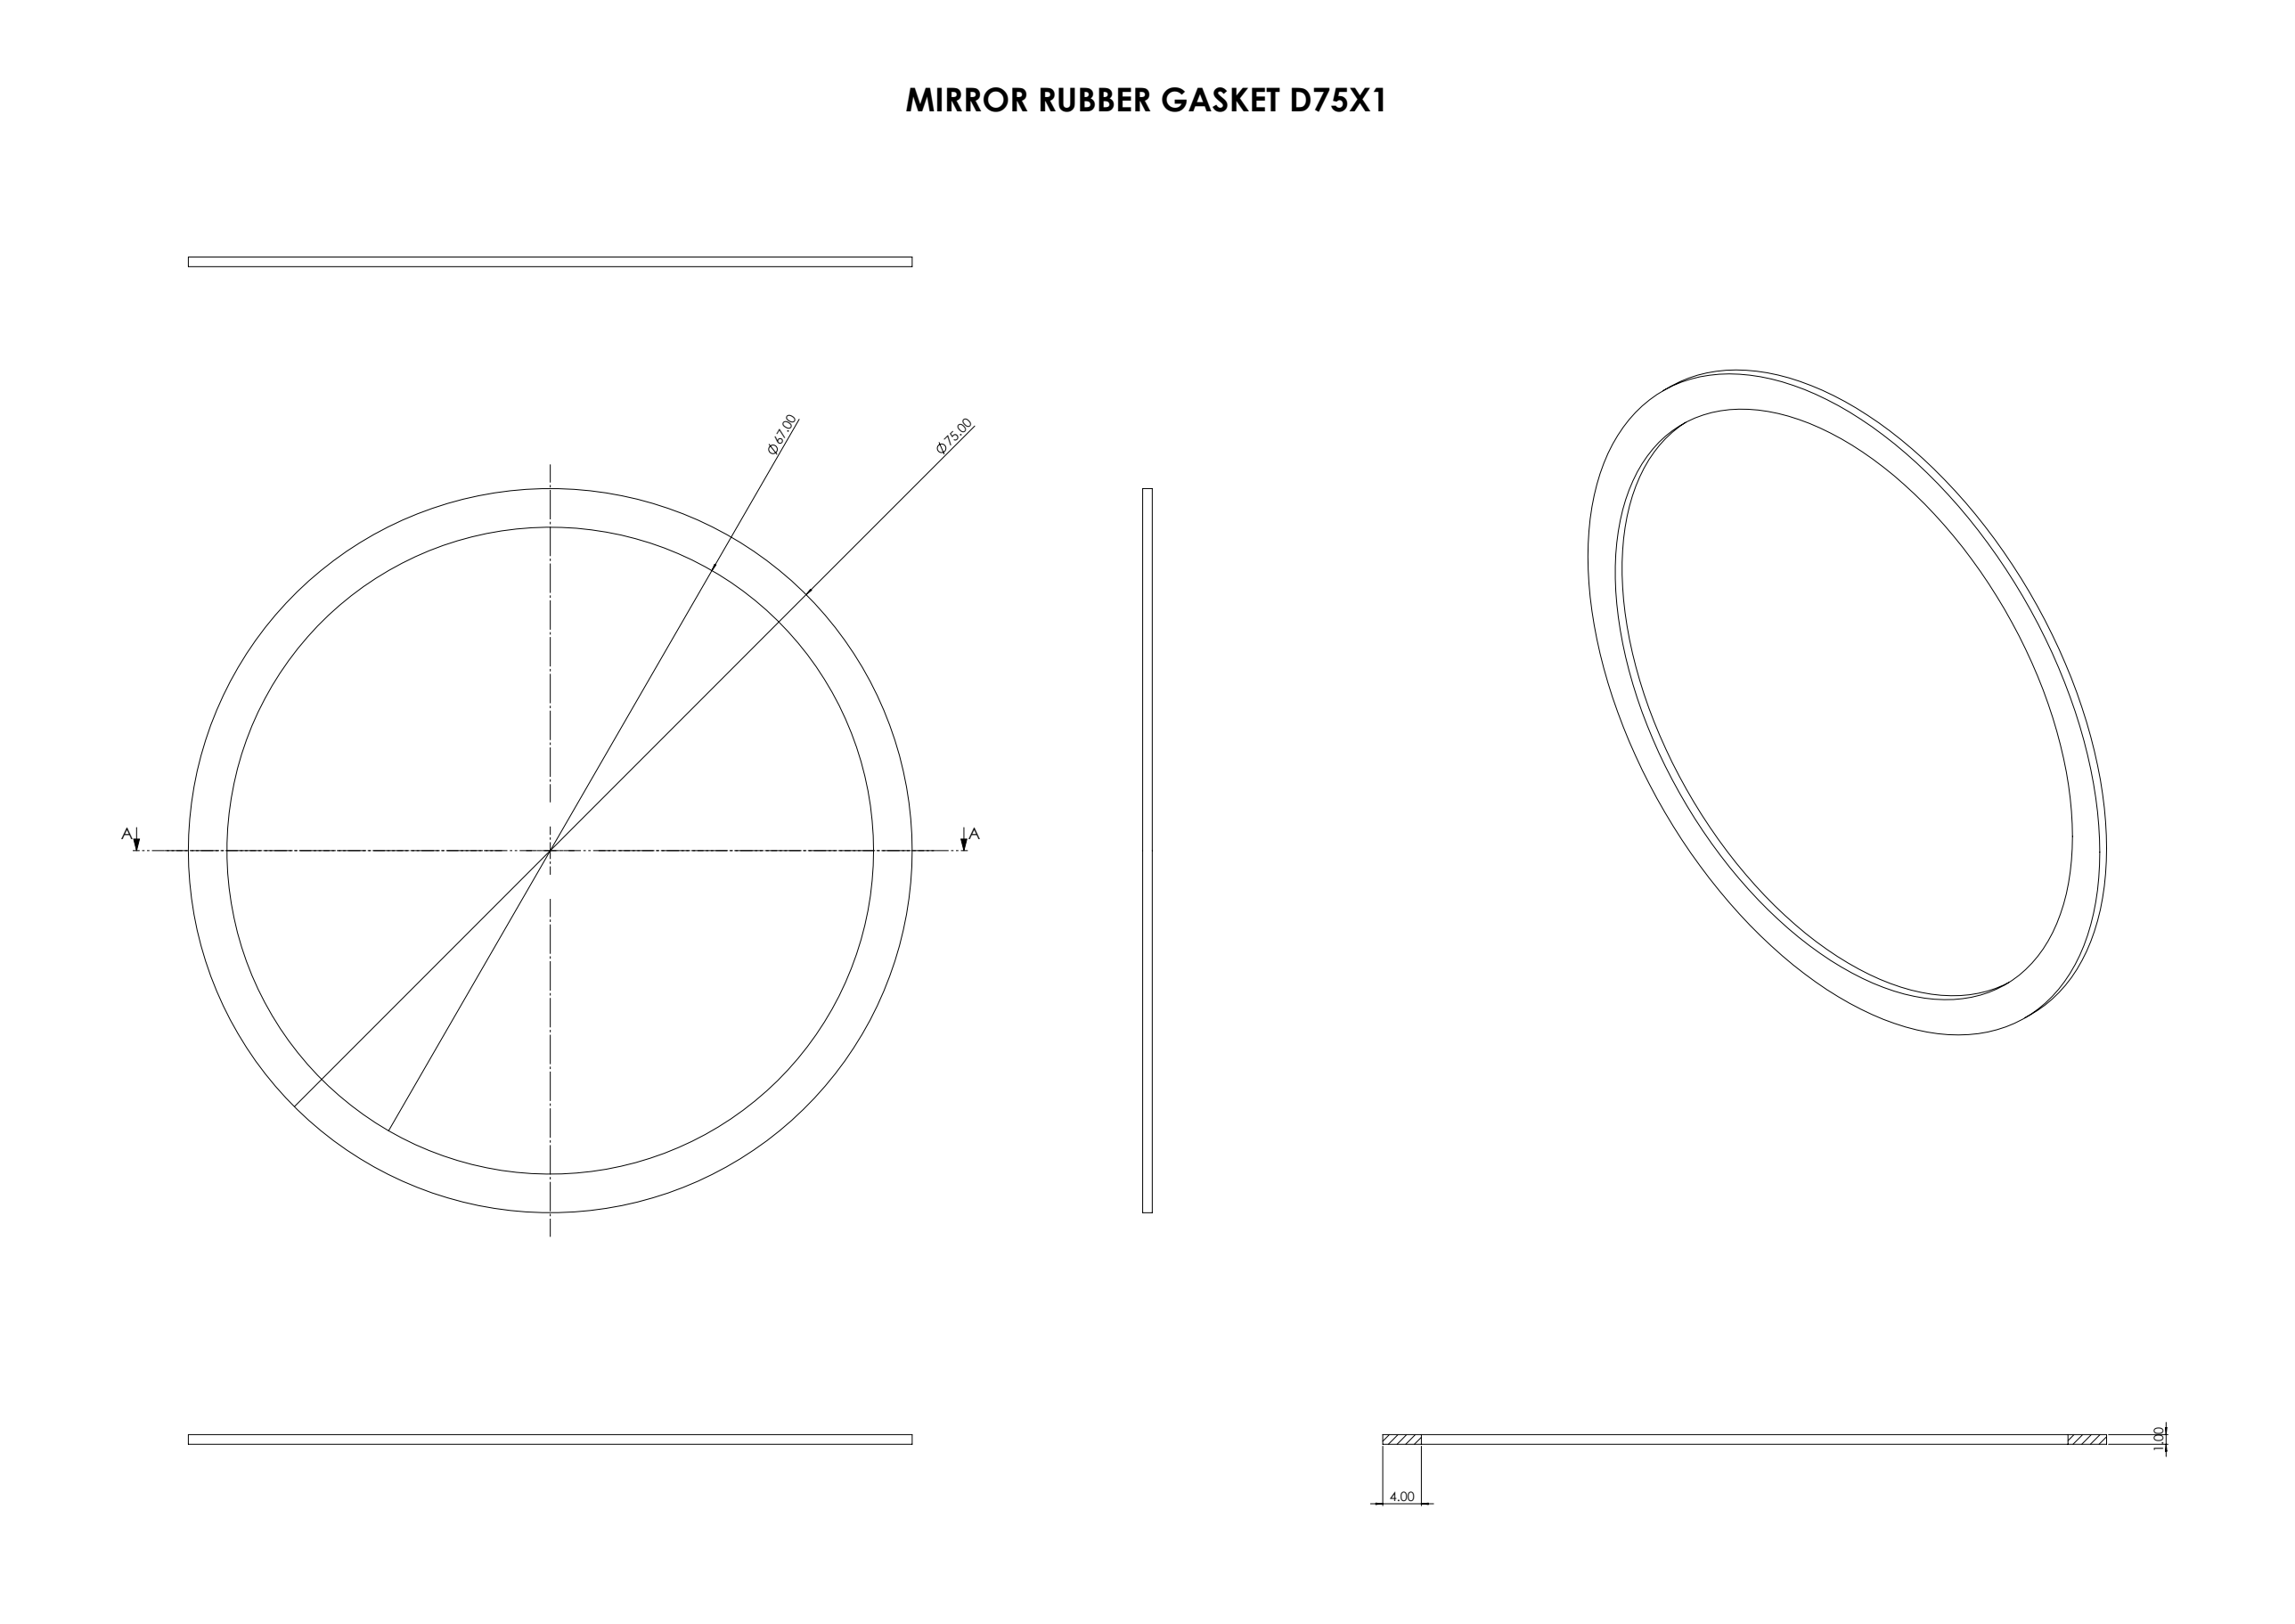
ISO-10303-21;
HEADER;
/* Generated by software containing ST-Developer
 * from STEP Tools, Inc. (www.steptools.com) 
 */

FILE_DESCRIPTION(
/* description */ (''),
/* implementation_level */ '2;1');

FILE_NAME(
/* name */ '08_Mirror_Rubber_Gasket_D75x1.step',
/* time_stamp */ '2026-10-19T22:59:19-07:00',
/* author */ (''),
/* organization */ (''),
/* preprocessor_version */ 'ST-DEVELOPER v20.2',
/* originating_system */ 'Autodesk Translation Framework v15.15.0.0',
/* authorisation */ '');

FILE_SCHEMA (('AUTOMOTIVE_DESIGN { 1 0 10303 214 3 1 1 }'));
ENDSEC;

DATA;
#10=MECHANICAL_DESIGN_GEOMETRIC_PRESENTATION_REPRESENTATION('',(#920),#53650);
#888=SHAPE_REPRESENTATION_RELATIONSHIP('SRR','None',#53733,#904);
#904=ADVANCED_BREP_SHAPE_REPRESENTATION('',(#936),#53643);
#920=STYLED_ITEM('',(#53965),#936);
#936=MANIFOLD_SOLID_BREP('Gasket',#23312);
#1044=CYLINDRICAL_SURFACE('',#24522,3.35);
#1045=CYLINDRICAL_SURFACE('',#24527,3.75);
#1410=FACE_BOUND('',#4277,.T.);
#1411=FACE_BOUND('',#4280,.T.);
#1755=PLANE('',#24525);
#1756=PLANE('',#24529);
#2814=FACE_OUTER_BOUND('',#4275,.T.);
#2815=FACE_OUTER_BOUND('',#4276,.T.);
#2816=FACE_OUTER_BOUND('',#4278,.T.);
#2817=FACE_OUTER_BOUND('',#4279,.T.);
#4275=EDGE_LOOP('',(#17615,#17616,#17617,#17618));
#4276=EDGE_LOOP('',(#17619));
#4277=EDGE_LOOP('',(#17620));
#4278=EDGE_LOOP('',(#17621,#17622,#17623,#17624));
#4279=EDGE_LOOP('',(#17625));
#4280=EDGE_LOOP('',(#17626));
#5502=CIRCLE('',#24523,3.35);
#5503=CIRCLE('',#24524,3.35);
#5504=CIRCLE('',#24526,3.75);
#5505=CIRCLE('',#24528,3.75);
#6636=LINE('',#35972,#8481);
#6637=LINE('',#35980,#8482);
#8481=VECTOR('',#28494,3.35);
#8482=VECTOR('',#28505,3.75);
#10333=VERTEX_POINT('',#35969);
#10334=VERTEX_POINT('',#35971);
#10335=VERTEX_POINT('',#35975);
#10336=VERTEX_POINT('',#35978);
#12985=EDGE_CURVE('',#10333,#10333,#5502,.T.);
#12986=EDGE_CURVE('',#10333,#10334,#6636,.T.);
#12987=EDGE_CURVE('',#10334,#10334,#5503,.T.);
#12988=EDGE_CURVE('',#10335,#10335,#5504,.T.);
#12989=EDGE_CURVE('',#10336,#10336,#5505,.T.);
#12990=EDGE_CURVE('',#10336,#10335,#6637,.T.);
#17615=ORIENTED_EDGE('',*,*,#12985,.T.);
#17616=ORIENTED_EDGE('',*,*,#12986,.T.);
#17617=ORIENTED_EDGE('',*,*,#12987,.F.);
#17618=ORIENTED_EDGE('',*,*,#12986,.F.);
#17619=ORIENTED_EDGE('',*,*,#12988,.F.);
#17620=ORIENTED_EDGE('',*,*,#12987,.T.);
#17621=ORIENTED_EDGE('',*,*,#12989,.F.);
#17622=ORIENTED_EDGE('',*,*,#12990,.T.);
#17623=ORIENTED_EDGE('',*,*,#12988,.T.);
#17624=ORIENTED_EDGE('',*,*,#12990,.F.);
#17625=ORIENTED_EDGE('',*,*,#12989,.T.);
#17626=ORIENTED_EDGE('',*,*,#12985,.F.);
#22553=ADVANCED_FACE('',(#2814),#1044,.F.);
#22554=ADVANCED_FACE('',(#2815,#1410),#1755,.T.);
#22555=ADVANCED_FACE('',(#2816),#1045,.T.);
#22556=ADVANCED_FACE('',(#2817,#1411),#1756,.T.);
#23312=CLOSED_SHELL('',(#22553,#22554,#22555,#22556));
#24521=AXIS2_PLACEMENT_3D('',#35967,#28488,#28489);
#24522=AXIS2_PLACEMENT_3D('',#35968,#28490,#28491);
#24523=AXIS2_PLACEMENT_3D('',#35970,#28492,#28493);
#24524=AXIS2_PLACEMENT_3D('',#35973,#28495,#28496);
#24525=AXIS2_PLACEMENT_3D('',#35974,#28497,#28498);
#24526=AXIS2_PLACEMENT_3D('',#35976,#28499,#28500);
#24527=AXIS2_PLACEMENT_3D('',#35977,#28501,#28502);
#24528=AXIS2_PLACEMENT_3D('',#35979,#28503,#28504);
#24529=AXIS2_PLACEMENT_3D('',#35981,#28506,#28507);
#28488=DIRECTION('axis',(0.,0.,1.));
#28489=DIRECTION('refdir',(1.,0.,0.));
#28490=DIRECTION('center_axis',(0.,0.,1.));
#28491=DIRECTION('ref_axis',(1.,0.,0.));
#28492=DIRECTION('center_axis',(0.,0.,1.));
#28493=DIRECTION('ref_axis',(1.,0.,0.));
#28494=DIRECTION('',(0.,0.,-1.));
#28495=DIRECTION('center_axis',(0.,0.,1.));
#28496=DIRECTION('ref_axis',(1.,0.,0.));
#28497=DIRECTION('center_axis',(0.,0.,-1.));
#28498=DIRECTION('ref_axis',(-1.,0.,0.));
#28499=DIRECTION('center_axis',(0.,0.,1.));
#28500=DIRECTION('ref_axis',(1.,0.,0.));
#28501=DIRECTION('center_axis',(0.,0.,1.));
#28502=DIRECTION('ref_axis',(1.,0.,0.));
#28503=DIRECTION('center_axis',(0.,0.,1.));
#28504=DIRECTION('ref_axis',(1.,0.,0.));
#28505=DIRECTION('',(0.,0.,-1.));
#28506=DIRECTION('center_axis',(0.,0.,1.));
#28507=DIRECTION('ref_axis',(1.,0.,0.));
#35967=CARTESIAN_POINT('',(0.,0.,0.));
#35968=CARTESIAN_POINT('Origin',(0.,0.,0.05));
#35969=CARTESIAN_POINT('',(-3.35,-4.10256677714363E-16,0.1));
#35970=CARTESIAN_POINT('Origin',(0.,0.,0.1));
#35971=CARTESIAN_POINT('',(-3.35,-4.10256677714363E-16,0.));
#35972=CARTESIAN_POINT('',(-3.35,-4.10256677714363E-16,0.05));
#35973=CARTESIAN_POINT('Origin',(0.,0.,0.));
#35974=CARTESIAN_POINT('Origin',(3.75,0.,0.));
#35975=CARTESIAN_POINT('',(-3.75,-4.59242549680257E-16,0.));
#35976=CARTESIAN_POINT('Origin',(0.,0.,0.));
#35977=CARTESIAN_POINT('Origin',(0.,0.,0.05));
#35978=CARTESIAN_POINT('',(-3.75,-4.59242549680257E-16,0.1));
#35979=CARTESIAN_POINT('Origin',(0.,0.,0.1));
#35980=CARTESIAN_POINT('',(-3.75,-4.59242549680257E-16,0.05));
#35981=CARTESIAN_POINT('Origin',(3.35,0.,0.1));
#53625=UNCERTAINTY_MEASURE_WITH_UNIT(LENGTH_MEASURE(0.001),#53651,
'DISTANCE_ACCURACY_VALUE',
'Maximum model space distance between geometric entities at asserted c
onnectivities');
#53632=UNCERTAINTY_MEASURE_WITH_UNIT(LENGTH_MEASURE(0.001),#53651,
'DISTANCE_ACCURACY_VALUE',
'Maximum model space distance between geometric entities at asserted c
onnectivities');
#53643=(
GEOMETRIC_REPRESENTATION_CONTEXT(3)
GLOBAL_UNCERTAINTY_ASSIGNED_CONTEXT((#53625))
GLOBAL_UNIT_ASSIGNED_CONTEXT((#53651,#53653,#53654))
REPRESENTATION_CONTEXT('','3D')
);
#53650=(
GEOMETRIC_REPRESENTATION_CONTEXT(3)
GLOBAL_UNCERTAINTY_ASSIGNED_CONTEXT((#53632))
GLOBAL_UNIT_ASSIGNED_CONTEXT((#53651,#53653,#53654))
REPRESENTATION_CONTEXT('','3D')
);
#53651=(
LENGTH_UNIT()
NAMED_UNIT(*)
SI_UNIT(.CENTI.,.METRE.)
);
#53653=(
NAMED_UNIT(*)
PLANE_ANGLE_UNIT()
SI_UNIT($,.RADIAN.)
);
#53654=(
NAMED_UNIT(*)
SI_UNIT($,.STERADIAN.)
SOLID_ANGLE_UNIT()
);
#53665=SHAPE_DEFINITION_REPRESENTATION(#53682,#53733);
#53682=PRODUCT_DEFINITION_SHAPE('',$,#53751);
#53733=SHAPE_REPRESENTATION('',(#24521),#53643);
#53740=PRODUCT_DEFINITION_CONTEXT('part definition',#53793,'design');
#53751=PRODUCT_DEFINITION('2026-10-18-22-44-43-283',
'08_Mirror_Rubber_Gasket_D75x1',#53768,#53740);
#53768=PRODUCT_DEFINITION_FORMATION('',$,#53805);
#53793=APPLICATION_CONTEXT(
'Core Data for Automotive Mechanical Design Process');
#53794=PRODUCT_CONTEXT('part definition',#53793,'mechanical');
#53805=PRODUCT('2026-10-18-22-44-43-283',
'08_Mirror_Rubber_Gasket_D75x1',$,(#53794));
#53959=COLOUR_RGB('Black',0.12,0.14,0.17);
#53960=FILL_AREA_STYLE_COLOUR('',#53959);
#53961=FILL_AREA_STYLE('',(#53960));
#53962=SURFACE_STYLE_FILL_AREA(#53961);
#53963=SURFACE_SIDE_STYLE('',(#53962));
#53964=SURFACE_STYLE_USAGE(.BOTH.,#53963);
#53965=PRESENTATION_STYLE_ASSIGNMENT((#53964));
ENDSEC;
END-ISO-10303-21;
